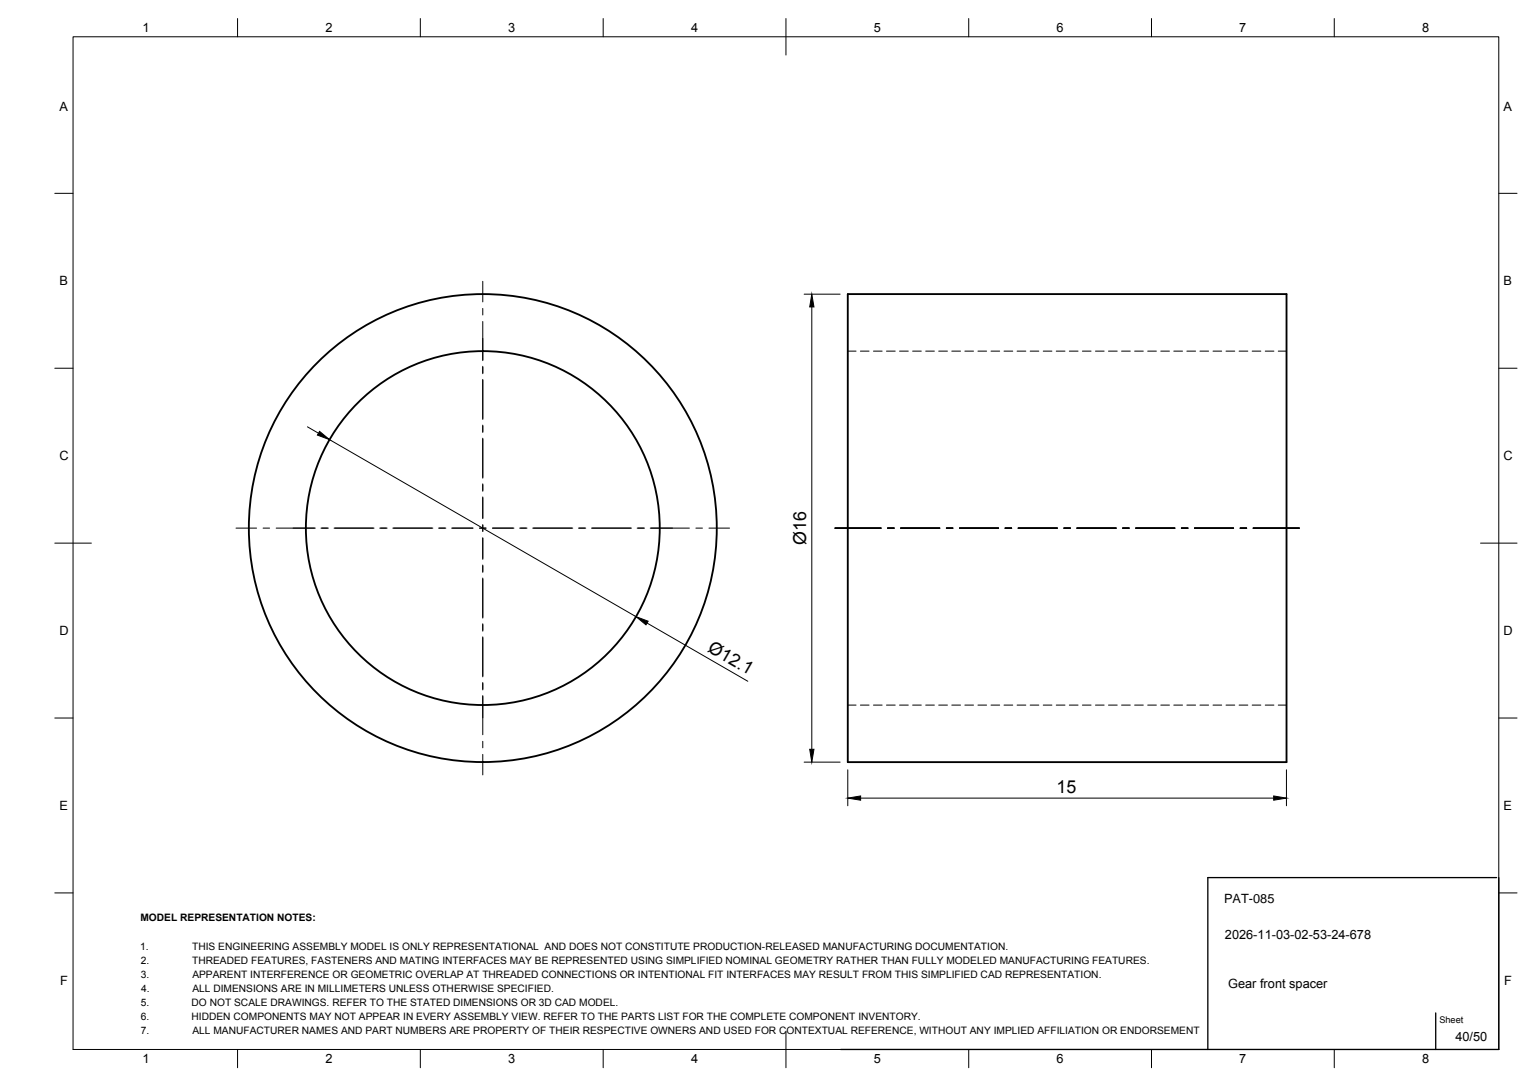
ISO-10303-21;
HEADER;
/* Generated by software containing ST-Developer
 * from STEP Tools, Inc. (www.steptools.com) 
 */

FILE_DESCRIPTION(
/* description */ ('Rack and pinion manual slide'),
/* implementation_level */ '2;1');

FILE_NAME(
/* name */ 'Gear front spacer.step',
/* time_stamp */ '2026-10-28T03:22:49-07:00',
/* author */ (''),
/* organization */ (''),
/* preprocessor_version */ 'ST-DEVELOPER v20.2',
/* originating_system */ 'Autodesk Translation Framework v15.17.0.0',
/* authorisation */ '');

FILE_SCHEMA (('AUTOMOTIVE_DESIGN { 1 0 10303 214 3 1 1 }'));
ENDSEC;

DATA;
#10=MECHANICAL_DESIGN_GEOMETRIC_PRESENTATION_REPRESENTATION('',(#771),#34851);
#672=SHAPE_REPRESENTATION_RELATIONSHIP('SRR','None',#35111,#718);
#718=ADVANCED_BREP_SHAPE_REPRESENTATION('',(#821),#34836);
#771=STYLED_ITEM('',(#35404),#821);
#821=MANIFOLD_SOLID_BREP('Body1',#13794);
#1016=FACE_BOUND('',#3018,.T.);
#1017=FACE_BOUND('',#3020,.T.);
#1450=PLANE('',#15242);
#1451=PLANE('',#15243);
#2093=FACE_OUTER_BOUND('',#3015,.T.);
#2094=FACE_OUTER_BOUND('',#3016,.T.);
#2095=FACE_OUTER_BOUND('',#3017,.T.);
#2096=FACE_OUTER_BOUND('',#3019,.T.);
#3015=EDGE_LOOP('',(#11990,#11991,#11992,#11993));
#3016=EDGE_LOOP('',(#11994,#11995,#11996,#11997));
#3017=EDGE_LOOP('',(#11998));
#3018=EDGE_LOOP('',(#11999));
#3019=EDGE_LOOP('',(#12000));
#3020=EDGE_LOOP('',(#12001));
#4274=LINE('',#22661,#5565);
#4275=LINE('',#22667,#5566);
#5565=VECTOR('',#18492,0.605);
#5566=VECTOR('',#18499,0.800000000000001);
#6118=CIRCLE('',#15237,0.605);
#6119=CIRCLE('',#15238,0.605);
#6120=CIRCLE('',#15240,0.800000000000001);
#6121=CIRCLE('',#15241,0.800000000000001);
#7147=VERTEX_POINT('',#22658);
#7148=VERTEX_POINT('',#22660);
#7149=VERTEX_POINT('',#22664);
#7150=VERTEX_POINT('',#22666);
#8807=EDGE_CURVE('',#7147,#7147,#6118,.T.);
#8808=EDGE_CURVE('',#7147,#7148,#4274,.T.);
#8809=EDGE_CURVE('',#7148,#7148,#6119,.T.);
#8810=EDGE_CURVE('',#7149,#7149,#6120,.T.);
#8811=EDGE_CURVE('',#7149,#7150,#4275,.T.);
#8812=EDGE_CURVE('',#7150,#7150,#6121,.T.);
#11990=ORIENTED_EDGE('',*,*,#8807,.F.);
#11991=ORIENTED_EDGE('',*,*,#8808,.T.);
#11992=ORIENTED_EDGE('',*,*,#8809,.T.);
#11993=ORIENTED_EDGE('',*,*,#8808,.F.);
#11994=ORIENTED_EDGE('',*,*,#8810,.F.);
#11995=ORIENTED_EDGE('',*,*,#8811,.T.);
#11996=ORIENTED_EDGE('',*,*,#8812,.T.);
#11997=ORIENTED_EDGE('',*,*,#8811,.F.);
#11998=ORIENTED_EDGE('',*,*,#8810,.T.);
#11999=ORIENTED_EDGE('',*,*,#8807,.T.);
#12000=ORIENTED_EDGE('',*,*,#8812,.F.);
#12001=ORIENTED_EDGE('',*,*,#8809,.F.);
#12965=CYLINDRICAL_SURFACE('',#15236,0.605);
#12966=CYLINDRICAL_SURFACE('',#15239,0.800000000000001);
#13571=ADVANCED_FACE('',(#2093),#12965,.F.);
#13572=ADVANCED_FACE('',(#2094),#12966,.T.);
#13573=ADVANCED_FACE('',(#2095,#1016),#1450,.T.);
#13574=ADVANCED_FACE('',(#2096,#1017),#1451,.F.);
#13794=CLOSED_SHELL('',(#13571,#13572,#13573,#13574));
#15235=AXIS2_PLACEMENT_3D('',#22656,#18486,#18487);
#15236=AXIS2_PLACEMENT_3D('',#22657,#18488,#18489);
#15237=AXIS2_PLACEMENT_3D('',#22659,#18490,#18491);
#15238=AXIS2_PLACEMENT_3D('',#22662,#18493,#18494);
#15239=AXIS2_PLACEMENT_3D('',#22663,#18495,#18496);
#15240=AXIS2_PLACEMENT_3D('',#22665,#18497,#18498);
#15241=AXIS2_PLACEMENT_3D('',#22668,#18500,#18501);
#15242=AXIS2_PLACEMENT_3D('',#22669,#18502,#18503);
#15243=AXIS2_PLACEMENT_3D('',#22670,#18504,#18505);
#18486=DIRECTION('axis',(0.,0.,1.));
#18487=DIRECTION('refdir',(1.,0.,0.));
#18488=DIRECTION('center_axis',(0.,1.,0.));
#18489=DIRECTION('ref_axis',(1.,0.,0.));
#18490=DIRECTION('center_axis',(0.,-1.,0.));
#18491=DIRECTION('ref_axis',(1.,0.,0.));
#18492=DIRECTION('',(0.,-1.,0.));
#18493=DIRECTION('center_axis',(0.,-1.,0.));
#18494=DIRECTION('ref_axis',(1.,0.,0.));
#18495=DIRECTION('center_axis',(0.,1.,0.));
#18496=DIRECTION('ref_axis',(1.,0.,0.));
#18497=DIRECTION('center_axis',(0.,1.,0.));
#18498=DIRECTION('ref_axis',(1.,0.,0.));
#18499=DIRECTION('',(0.,-1.,0.));
#18500=DIRECTION('center_axis',(0.,1.,0.));
#18501=DIRECTION('ref_axis',(1.,0.,0.));
#18502=DIRECTION('center_axis',(0.,1.,0.));
#18503=DIRECTION('ref_axis',(1.,0.,0.));
#18504=DIRECTION('center_axis',(0.,1.,0.));
#18505=DIRECTION('ref_axis',(1.,0.,0.));
#22656=CARTESIAN_POINT('',(0.,0.,0.));
#22657=CARTESIAN_POINT('Origin',(11.,2.2,10.25));
#22658=CARTESIAN_POINT('',(10.395,3.7,10.25));
#22659=CARTESIAN_POINT('Origin',(11.,3.7,10.25));
#22660=CARTESIAN_POINT('',(10.395,2.2,10.25));
#22661=CARTESIAN_POINT('',(10.395,2.2,10.25));
#22662=CARTESIAN_POINT('Origin',(11.,2.2,10.25));
#22663=CARTESIAN_POINT('Origin',(11.,2.2,10.25));
#22664=CARTESIAN_POINT('',(10.2,3.7,10.25));
#22665=CARTESIAN_POINT('Origin',(11.,3.7,10.25));
#22666=CARTESIAN_POINT('',(10.2,2.2,10.25));
#22667=CARTESIAN_POINT('',(10.2,2.2,10.25));
#22668=CARTESIAN_POINT('Origin',(11.,2.2,10.25));
#22669=CARTESIAN_POINT('Origin',(11.,3.7,10.25));
#22670=CARTESIAN_POINT('Origin',(11.,2.2,10.25));
#34782=UNCERTAINTY_MEASURE_WITH_UNIT(LENGTH_MEASURE(0.001),#34852,
'DISTANCE_ACCURACY_VALUE',
'Maximum model space distance between geometric entities at asserted c
onnectivities');
#34797=UNCERTAINTY_MEASURE_WITH_UNIT(LENGTH_MEASURE(0.001),#34852,
'DISTANCE_ACCURACY_VALUE',
'Maximum model space distance between geometric entities at asserted c
onnectivities');
#34836=(
GEOMETRIC_REPRESENTATION_CONTEXT(3)
GLOBAL_UNCERTAINTY_ASSIGNED_CONTEXT((#34782))
GLOBAL_UNIT_ASSIGNED_CONTEXT((#34852,#34854,#34855))
REPRESENTATION_CONTEXT('','3D')
);
#34851=(
GEOMETRIC_REPRESENTATION_CONTEXT(3)
GLOBAL_UNCERTAINTY_ASSIGNED_CONTEXT((#34797))
GLOBAL_UNIT_ASSIGNED_CONTEXT((#34852,#34854,#34855))
REPRESENTATION_CONTEXT('','3D')
);
#34852=(
LENGTH_UNIT()
NAMED_UNIT(*)
SI_UNIT(.CENTI.,.METRE.)
);
#34854=(
NAMED_UNIT(*)
PLANE_ANGLE_UNIT()
SI_UNIT($,.RADIAN.)
);
#34855=(
NAMED_UNIT(*)
SI_UNIT($,.STERADIAN.)
SOLID_ANGLE_UNIT()
);
#34894=SHAPE_DEFINITION_REPRESENTATION(#34955,#35111);
#34955=PRODUCT_DEFINITION_SHAPE('',$,#35165);
#35111=SHAPE_REPRESENTATION('',(#15235),#34836);
#35126=PRODUCT_DEFINITION_CONTEXT('part definition',#35287,'design');
#35165=PRODUCT_DEFINITION('Gear front spacer','Gear front spacer',#35218,
#35126);
#35218=PRODUCT_DEFINITION_FORMATION('',$,#35327);
#35287=APPLICATION_CONTEXT(
'Core Data for Automotive Mechanical Design Process');
#35288=PRODUCT_CONTEXT('part definition',#35287,'mechanical');
#35327=PRODUCT('Gear front spacer','Gear front spacer',
'Gear front spacer',(#35288));
#35398=COLOUR_RGB('Sky Blue',0.24,0.69,0.87);
#35399=FILL_AREA_STYLE_COLOUR('',#35398);
#35400=FILL_AREA_STYLE('',(#35399));
#35401=SURFACE_STYLE_FILL_AREA(#35400);
#35402=SURFACE_SIDE_STYLE('',(#35401));
#35403=SURFACE_STYLE_USAGE(.BOTH.,#35402);
#35404=PRESENTATION_STYLE_ASSIGNMENT((#35403));
ENDSEC;
END-ISO-10303-21;
